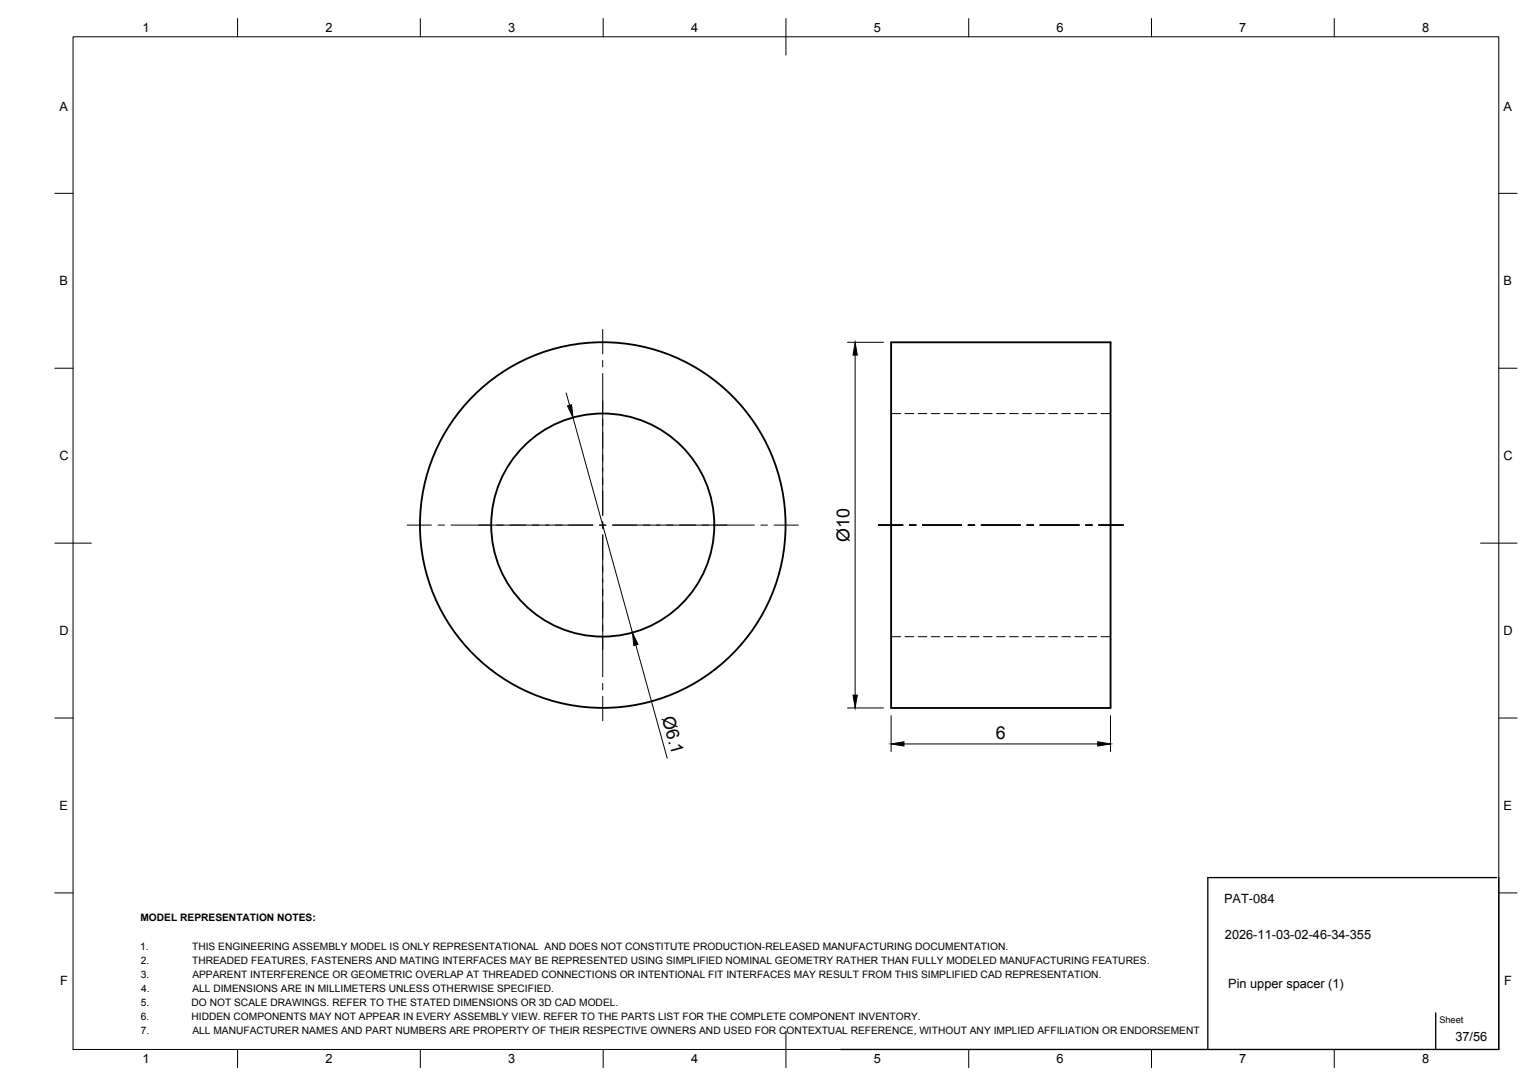
ISO-10303-21;
HEADER;
/* Generated by software containing ST-Developer
 * from STEP Tools, Inc. (www.steptools.com) 
 */

FILE_DESCRIPTION(
/* description */ ('Quick-return (Whitworth) mechanism'),
/* implementation_level */ '2;1');

FILE_NAME(
/* name */ 'Pin upper spacer (1).step',
/* time_stamp */ '2026-10-28T03:25:57-07:00',
/* author */ (''),
/* organization */ (''),
/* preprocessor_version */ 'ST-DEVELOPER v20.2',
/* originating_system */ 'Autodesk Translation Framework v15.17.0.0',
/* authorisation */ '');

FILE_SCHEMA (('AUTOMOTIVE_DESIGN { 1 0 10303 214 3 1 1 }'));
ENDSEC;

DATA;
#10=MECHANICAL_DESIGN_GEOMETRIC_PRESENTATION_REPRESENTATION('',(#525),#14878);
#429=SHAPE_REPRESENTATION_RELATIONSHIP('SRR','None',#15100,#473);
#473=ADVANCED_BREP_SHAPE_REPRESENTATION('',(#576),#14857);
#525=STYLED_ITEM('',(#15406),#576);
#576=MANIFOLD_SOLID_BREP('Body1',#7880);
#742=FACE_BOUND('',#1977,.T.);
#743=FACE_BOUND('',#1979,.T.);
#935=PLANE('',#9064);
#936=PLANE('',#9065);
#1357=FACE_OUTER_BOUND('',#1974,.T.);
#1358=FACE_OUTER_BOUND('',#1975,.T.);
#1359=FACE_OUTER_BOUND('',#1976,.T.);
#1360=FACE_OUTER_BOUND('',#1978,.T.);
#1974=EDGE_LOOP('',(#6528,#6529,#6530,#6531));
#1975=EDGE_LOOP('',(#6532,#6533,#6534,#6535));
#1976=EDGE_LOOP('',(#6536));
#1977=EDGE_LOOP('',(#6537));
#1978=EDGE_LOOP('',(#6538));
#1979=EDGE_LOOP('',(#6539));
#2441=LINE('',#13959,#2964);
#2442=LINE('',#13965,#2965);
#2964=VECTOR('',#11020,0.305);
#2965=VECTOR('',#11027,0.5);
#3542=CIRCLE('',#9059,0.305);
#3543=CIRCLE('',#9060,0.305);
#3544=CIRCLE('',#9062,0.5);
#3545=CIRCLE('',#9063,0.5);
#4063=VERTEX_POINT('',#13956);
#4064=VERTEX_POINT('',#13958);
#4065=VERTEX_POINT('',#13962);
#4066=VERTEX_POINT('',#13964);
#4921=EDGE_CURVE('',#4063,#4063,#3542,.T.);
#4922=EDGE_CURVE('',#4063,#4064,#2441,.T.);
#4923=EDGE_CURVE('',#4064,#4064,#3543,.T.);
#4924=EDGE_CURVE('',#4065,#4065,#3544,.T.);
#4925=EDGE_CURVE('',#4065,#4066,#2442,.T.);
#4926=EDGE_CURVE('',#4066,#4066,#3545,.T.);
#6528=ORIENTED_EDGE('',*,*,#4921,.F.);
#6529=ORIENTED_EDGE('',*,*,#4922,.T.);
#6530=ORIENTED_EDGE('',*,*,#4923,.T.);
#6531=ORIENTED_EDGE('',*,*,#4922,.F.);
#6532=ORIENTED_EDGE('',*,*,#4924,.F.);
#6533=ORIENTED_EDGE('',*,*,#4925,.T.);
#6534=ORIENTED_EDGE('',*,*,#4926,.T.);
#6535=ORIENTED_EDGE('',*,*,#4925,.F.);
#6536=ORIENTED_EDGE('',*,*,#4924,.T.);
#6537=ORIENTED_EDGE('',*,*,#4921,.T.);
#6538=ORIENTED_EDGE('',*,*,#4926,.F.);
#6539=ORIENTED_EDGE('',*,*,#4923,.F.);
#7341=CYLINDRICAL_SURFACE('',#9058,0.305);
#7342=CYLINDRICAL_SURFACE('',#9061,0.5);
#7688=ADVANCED_FACE('',(#1357),#7341,.F.);
#7689=ADVANCED_FACE('',(#1358),#7342,.T.);
#7690=ADVANCED_FACE('',(#1359,#742),#935,.T.);
#7691=ADVANCED_FACE('',(#1360,#743),#936,.F.);
#7880=CLOSED_SHELL('',(#7688,#7689,#7690,#7691));
#9057=AXIS2_PLACEMENT_3D('',#13954,#11014,#11015);
#9058=AXIS2_PLACEMENT_3D('',#13955,#11016,#11017);
#9059=AXIS2_PLACEMENT_3D('',#13957,#11018,#11019);
#9060=AXIS2_PLACEMENT_3D('',#13960,#11021,#11022);
#9061=AXIS2_PLACEMENT_3D('',#13961,#11023,#11024);
#9062=AXIS2_PLACEMENT_3D('',#13963,#11025,#11026);
#9063=AXIS2_PLACEMENT_3D('',#13966,#11028,#11029);
#9064=AXIS2_PLACEMENT_3D('',#13967,#11030,#11031);
#9065=AXIS2_PLACEMENT_3D('',#13968,#11032,#11033);
#11014=DIRECTION('axis',(0.,0.,1.));
#11015=DIRECTION('refdir',(1.,0.,0.));
#11016=DIRECTION('center_axis',(0.,0.,1.));
#11017=DIRECTION('ref_axis',(1.,0.,0.));
#11018=DIRECTION('center_axis',(0.,0.,-1.));
#11019=DIRECTION('ref_axis',(1.,0.,0.));
#11020=DIRECTION('',(0.,0.,-1.));
#11021=DIRECTION('center_axis',(0.,0.,-1.));
#11022=DIRECTION('ref_axis',(1.,0.,0.));
#11023=DIRECTION('center_axis',(0.,0.,1.));
#11024=DIRECTION('ref_axis',(1.,0.,0.));
#11025=DIRECTION('center_axis',(0.,0.,1.));
#11026=DIRECTION('ref_axis',(1.,0.,0.));
#11027=DIRECTION('',(0.,0.,-1.));
#11028=DIRECTION('center_axis',(0.,0.,1.));
#11029=DIRECTION('ref_axis',(1.,0.,0.));
#11030=DIRECTION('center_axis',(0.,0.,1.));
#11031=DIRECTION('ref_axis',(1.,0.,0.));
#11032=DIRECTION('center_axis',(0.,0.,1.));
#11033=DIRECTION('ref_axis',(1.,0.,0.));
#13954=CARTESIAN_POINT('',(0.,0.,0.));
#13955=CARTESIAN_POINT('Origin',(0.,12.,9.2));
#13956=CARTESIAN_POINT('',(-0.305,12.,9.8));
#13957=CARTESIAN_POINT('Origin',(0.,12.,9.8));
#13958=CARTESIAN_POINT('',(-0.305,12.,9.2));
#13959=CARTESIAN_POINT('',(-0.305,12.,9.2));
#13960=CARTESIAN_POINT('Origin',(0.,12.,9.2));
#13961=CARTESIAN_POINT('Origin',(0.,12.,9.2));
#13962=CARTESIAN_POINT('',(-0.5,12.,9.8));
#13963=CARTESIAN_POINT('Origin',(0.,12.,9.8));
#13964=CARTESIAN_POINT('',(-0.5,12.,9.2));
#13965=CARTESIAN_POINT('',(-0.5,12.,9.2));
#13966=CARTESIAN_POINT('Origin',(0.,12.,9.2));
#13967=CARTESIAN_POINT('Origin',(0.,12.,9.8));
#13968=CARTESIAN_POINT('Origin',(0.,12.,9.2));
#14803=UNCERTAINTY_MEASURE_WITH_UNIT(LENGTH_MEASURE(0.001),#14879,
'DISTANCE_ACCURACY_VALUE',
'Maximum model space distance between geometric entities at asserted c
onnectivities');
#14824=UNCERTAINTY_MEASURE_WITH_UNIT(LENGTH_MEASURE(0.001),#14879,
'DISTANCE_ACCURACY_VALUE',
'Maximum model space distance between geometric entities at asserted c
onnectivities');
#14857=(
GEOMETRIC_REPRESENTATION_CONTEXT(3)
GLOBAL_UNCERTAINTY_ASSIGNED_CONTEXT((#14803))
GLOBAL_UNIT_ASSIGNED_CONTEXT((#14879,#14881,#14882))
REPRESENTATION_CONTEXT('','3D')
);
#14878=(
GEOMETRIC_REPRESENTATION_CONTEXT(3)
GLOBAL_UNCERTAINTY_ASSIGNED_CONTEXT((#14824))
GLOBAL_UNIT_ASSIGNED_CONTEXT((#14879,#14881,#14882))
REPRESENTATION_CONTEXT('','3D')
);
#14879=(
LENGTH_UNIT()
NAMED_UNIT(*)
SI_UNIT(.CENTI.,.METRE.)
);
#14881=(
NAMED_UNIT(*)
PLANE_ANGLE_UNIT()
SI_UNIT($,.RADIAN.)
);
#14882=(
NAMED_UNIT(*)
SI_UNIT($,.STERADIAN.)
SOLID_ANGLE_UNIT()
);
#14915=SHAPE_DEFINITION_REPRESENTATION(#14973,#15100);
#14973=PRODUCT_DEFINITION_SHAPE('',$,#15154);
#15100=SHAPE_REPRESENTATION('',(#9057),#14857);
#15121=PRODUCT_DEFINITION_CONTEXT('part definition',#15282,'design');
#15154=PRODUCT_DEFINITION('Pin upper spacer (1)','Pin upper spacer (1)',#15207,
#15121);
#15207=PRODUCT_DEFINITION_FORMATION('',$,#15316);
#15282=APPLICATION_CONTEXT(
'Core Data for Automotive Mechanical Design Process');
#15283=PRODUCT_CONTEXT('part definition',#15282,'mechanical');
#15316=PRODUCT('Pin upper spacer (1)','Pin upper spacer (1)',
'Pin upper spacer (1)',(#15283));
#15400=COLOUR_RGB('Grey',0.48,0.52,0.57);
#15401=FILL_AREA_STYLE_COLOUR('',#15400);
#15402=FILL_AREA_STYLE('',(#15401));
#15403=SURFACE_STYLE_FILL_AREA(#15402);
#15404=SURFACE_SIDE_STYLE('',(#15403));
#15405=SURFACE_STYLE_USAGE(.BOTH.,#15404);
#15406=PRESENTATION_STYLE_ASSIGNMENT((#15405));
ENDSEC;
END-ISO-10303-21;
